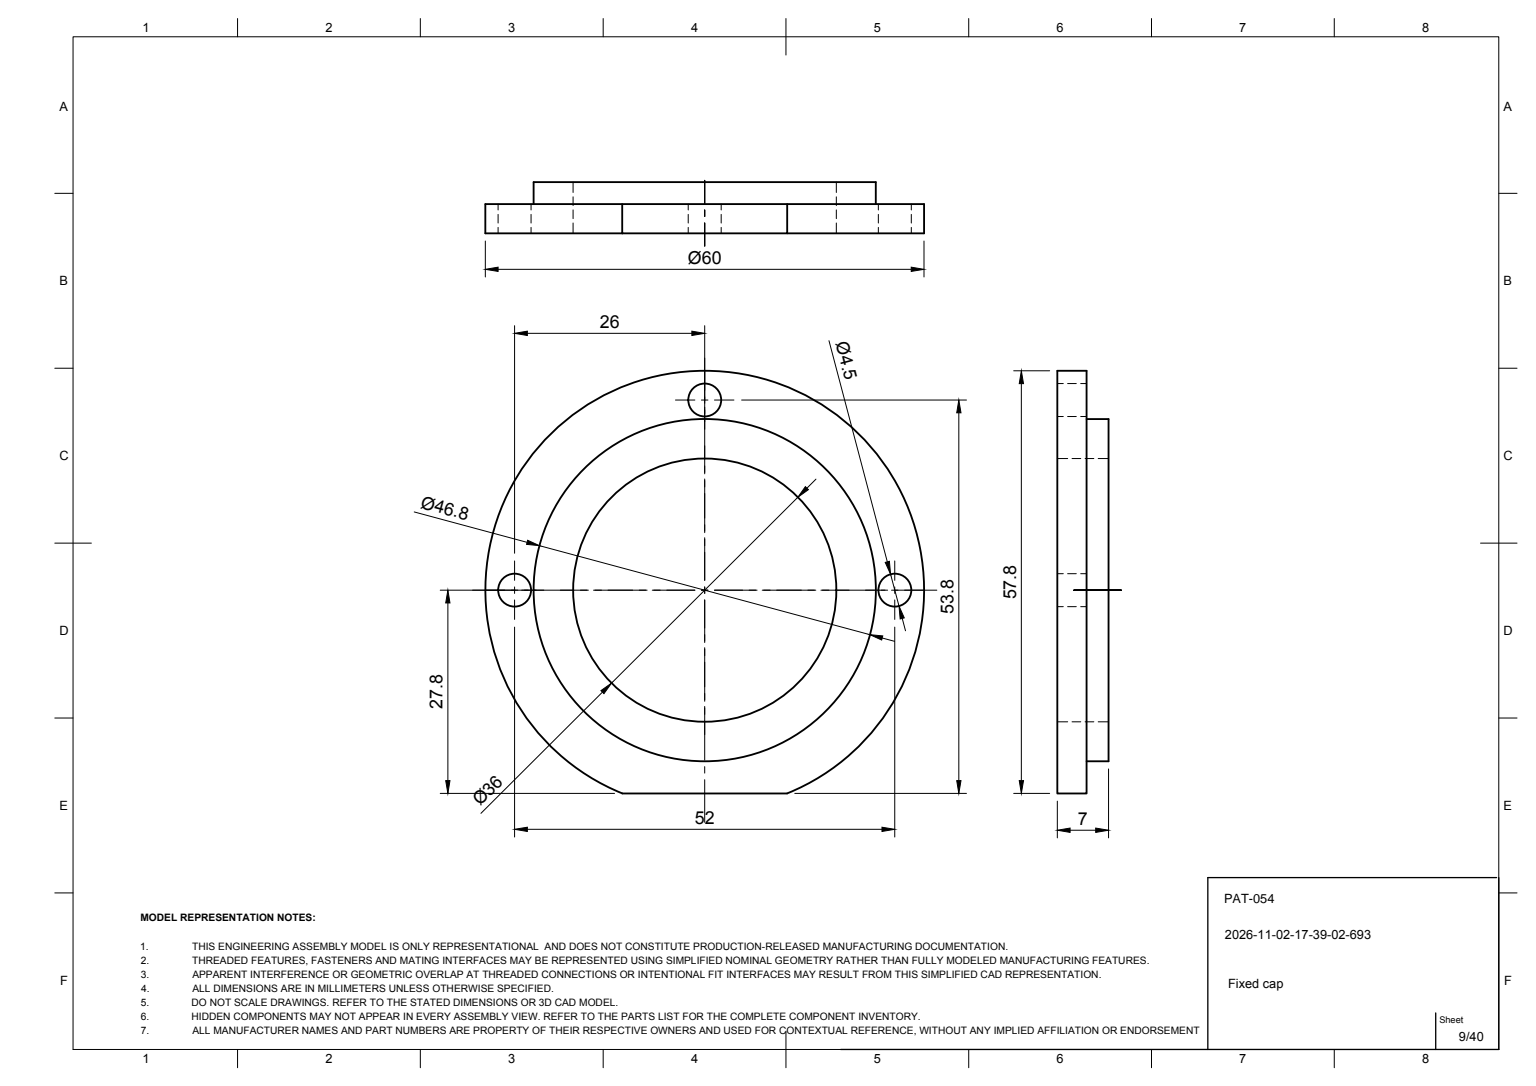
ISO-10303-21;
HEADER;
/* Generated by software containing ST-Developer
 * from STEP Tools, Inc. (www.steptools.com) 
 */

FILE_DESCRIPTION(
/* description */ ('PAT-054'),
/* implementation_level */ '2;1');

FILE_NAME(
/* name */ 'Fixed cap.step',
/* time_stamp */ '2026-10-29T16:38:13-07:00',
/* author */ (''),
/* organization */ (''),
/* preprocessor_version */ 'ST-DEVELOPER v20.2',
/* originating_system */ 'Autodesk Translation Framework v15.17.0.0',
/* authorisation */ '');

FILE_SCHEMA (('AUTOMOTIVE_DESIGN { 1 0 10303 214 3 1 1 }'));
ENDSEC;

DATA;
#10=MECHANICAL_DESIGN_GEOMETRIC_PRESENTATION_REPRESENTATION('',(#904),#33981);
#816=SHAPE_REPRESENTATION_RELATIONSHIP('SRR','None',#34189,#860);
#860=ADVANCED_BREP_SHAPE_REPRESENTATION('',(#963),#33937);
#904=STYLED_ITEM('',(#34531),#963);
#963=MANIFOLD_SOLID_BREP('Body1',#13015);
#1095=FACE_BOUND('',#2468,.T.);
#1096=FACE_BOUND('',#2469,.T.);
#1097=FACE_BOUND('',#2470,.T.);
#1098=FACE_BOUND('',#2471,.T.);
#1099=FACE_BOUND('',#2478,.T.);
#1100=FACE_BOUND('',#2481,.T.);
#1101=FACE_BOUND('',#2482,.T.);
#1102=FACE_BOUND('',#2483,.T.);
#1103=FACE_BOUND('',#2484,.T.);
#1265=PLANE('',#13748);
#1266=PLANE('',#13749);
#1267=PLANE('',#13765);
#1268=PLANE('',#13769);
#1660=FACE_OUTER_BOUND('',#2466,.T.);
#1661=FACE_OUTER_BOUND('',#2467,.T.);
#1662=FACE_OUTER_BOUND('',#2472,.T.);
#1663=FACE_OUTER_BOUND('',#2473,.T.);
#1664=FACE_OUTER_BOUND('',#2474,.T.);
#1665=FACE_OUTER_BOUND('',#2475,.T.);
#1666=FACE_OUTER_BOUND('',#2476,.T.);
#1667=FACE_OUTER_BOUND('',#2477,.T.);
#1668=FACE_OUTER_BOUND('',#2479,.T.);
#1669=FACE_OUTER_BOUND('',#2480,.T.);
#2466=EDGE_LOOP('',(#8873,#8874,#8875,#8876));
#2467=EDGE_LOOP('',(#8877,#8878));
#2468=EDGE_LOOP('',(#8879));
#2469=EDGE_LOOP('',(#8880));
#2470=EDGE_LOOP('',(#8881));
#2471=EDGE_LOOP('',(#8882));
#2472=EDGE_LOOP('',(#8883,#8884,#8885,#8886));
#2473=EDGE_LOOP('',(#8887,#8888,#8889,#8890));
#2474=EDGE_LOOP('',(#8891,#8892,#8893,#8894));
#2475=EDGE_LOOP('',(#8895,#8896,#8897,#8898));
#2476=EDGE_LOOP('',(#8899,#8900,#8901,#8902));
#2477=EDGE_LOOP('',(#8903));
#2478=EDGE_LOOP('',(#8904));
#2479=EDGE_LOOP('',(#8905,#8906,#8907,#8908));
#2480=EDGE_LOOP('',(#8909,#8910));
#2481=EDGE_LOOP('',(#8911));
#2482=EDGE_LOOP('',(#8912));
#2483=EDGE_LOOP('',(#8913));
#2484=EDGE_LOOP('',(#8914));
#3333=LINE('',#18902,#4267);
#3334=LINE('',#18904,#4268);
#3335=LINE('',#18906,#4269);
#3336=LINE('',#18907,#4270);
#3337=LINE('',#18922,#4271);
#3338=LINE('',#18926,#4272);
#3339=LINE('',#18930,#4273);
#3340=LINE('',#18934,#4274);
#3341=LINE('',#18942,#4275);
#4267=VECTOR('',#15366,1.);
#4268=VECTOR('',#15367,1.);
#4269=VECTOR('',#15368,1.);
#4270=VECTOR('',#15369,1.);
#4271=VECTOR('',#15388,0.225);
#4272=VECTOR('',#15393,0.225);
#4273=VECTOR('',#15398,0.225);
#4274=VECTOR('',#15403,2.34);
#4275=VECTOR('',#15414,1.8);
#5201=CIRCLE('',#13750,3.);
#5202=CIRCLE('',#13751,2.34);
#5203=CIRCLE('',#13752,0.225);
#5204=CIRCLE('',#13753,0.225);
#5205=CIRCLE('',#13754,0.225);
#5206=CIRCLE('',#13756,3.);
#5207=CIRCLE('',#13758,0.225);
#5208=CIRCLE('',#13760,0.225);
#5209=CIRCLE('',#13762,0.225);
#5210=CIRCLE('',#13764,2.34);
#5211=CIRCLE('',#13766,1.8);
#5212=CIRCLE('',#13768,1.8);
#5698=VERTEX_POINT('',#18900);
#5699=VERTEX_POINT('',#18901);
#5700=VERTEX_POINT('',#18903);
#5701=VERTEX_POINT('',#18905);
#5702=VERTEX_POINT('',#18910);
#5703=VERTEX_POINT('',#18912);
#5704=VERTEX_POINT('',#18914);
#5705=VERTEX_POINT('',#18916);
#5706=VERTEX_POINT('',#18921);
#5707=VERTEX_POINT('',#18925);
#5708=VERTEX_POINT('',#18929);
#5709=VERTEX_POINT('',#18933);
#5710=VERTEX_POINT('',#18937);
#5711=VERTEX_POINT('',#18940);
#6936=EDGE_CURVE('',#5698,#5699,#3333,.T.);
#6937=EDGE_CURVE('',#5700,#5698,#3334,.T.);
#6938=EDGE_CURVE('',#5701,#5700,#3335,.T.);
#6939=EDGE_CURVE('',#5699,#5701,#3336,.T.);
#6940=EDGE_CURVE('',#5700,#5698,#5201,.T.);
#6941=EDGE_CURVE('',#5702,#5702,#5202,.T.);
#6942=EDGE_CURVE('',#5703,#5703,#5203,.T.);
#6943=EDGE_CURVE('',#5704,#5704,#5204,.T.);
#6944=EDGE_CURVE('',#5705,#5705,#5205,.T.);
#6945=EDGE_CURVE('',#5701,#5699,#5206,.T.);
#6946=EDGE_CURVE('',#5705,#5706,#3337,.T.);
#6947=EDGE_CURVE('',#5706,#5706,#5207,.T.);
#6948=EDGE_CURVE('',#5704,#5707,#3338,.T.);
#6949=EDGE_CURVE('',#5707,#5707,#5208,.T.);
#6950=EDGE_CURVE('',#5703,#5708,#3339,.T.);
#6951=EDGE_CURVE('',#5708,#5708,#5209,.T.);
#6952=EDGE_CURVE('',#5702,#5709,#3340,.T.);
#6953=EDGE_CURVE('',#5709,#5709,#5210,.T.);
#6954=EDGE_CURVE('',#5710,#5710,#5211,.T.);
#6955=EDGE_CURVE('',#5711,#5711,#5212,.T.);
#6956=EDGE_CURVE('',#5711,#5710,#3341,.T.);
#8873=ORIENTED_EDGE('',*,*,#6936,.F.);
#8874=ORIENTED_EDGE('',*,*,#6937,.F.);
#8875=ORIENTED_EDGE('',*,*,#6938,.F.);
#8876=ORIENTED_EDGE('',*,*,#6939,.F.);
#8877=ORIENTED_EDGE('',*,*,#6937,.T.);
#8878=ORIENTED_EDGE('',*,*,#6940,.F.);
#8879=ORIENTED_EDGE('',*,*,#6941,.T.);
#8880=ORIENTED_EDGE('',*,*,#6942,.T.);
#8881=ORIENTED_EDGE('',*,*,#6943,.T.);
#8882=ORIENTED_EDGE('',*,*,#6944,.T.);
#8883=ORIENTED_EDGE('',*,*,#6938,.T.);
#8884=ORIENTED_EDGE('',*,*,#6940,.T.);
#8885=ORIENTED_EDGE('',*,*,#6936,.T.);
#8886=ORIENTED_EDGE('',*,*,#6945,.F.);
#8887=ORIENTED_EDGE('',*,*,#6944,.F.);
#8888=ORIENTED_EDGE('',*,*,#6946,.T.);
#8889=ORIENTED_EDGE('',*,*,#6947,.F.);
#8890=ORIENTED_EDGE('',*,*,#6946,.F.);
#8891=ORIENTED_EDGE('',*,*,#6943,.F.);
#8892=ORIENTED_EDGE('',*,*,#6948,.T.);
#8893=ORIENTED_EDGE('',*,*,#6949,.F.);
#8894=ORIENTED_EDGE('',*,*,#6948,.F.);
#8895=ORIENTED_EDGE('',*,*,#6942,.F.);
#8896=ORIENTED_EDGE('',*,*,#6950,.T.);
#8897=ORIENTED_EDGE('',*,*,#6951,.F.);
#8898=ORIENTED_EDGE('',*,*,#6950,.F.);
#8899=ORIENTED_EDGE('',*,*,#6941,.F.);
#8900=ORIENTED_EDGE('',*,*,#6952,.T.);
#8901=ORIENTED_EDGE('',*,*,#6953,.T.);
#8902=ORIENTED_EDGE('',*,*,#6952,.F.);
#8903=ORIENTED_EDGE('',*,*,#6953,.F.);
#8904=ORIENTED_EDGE('',*,*,#6954,.F.);
#8905=ORIENTED_EDGE('',*,*,#6955,.F.);
#8906=ORIENTED_EDGE('',*,*,#6956,.T.);
#8907=ORIENTED_EDGE('',*,*,#6954,.T.);
#8908=ORIENTED_EDGE('',*,*,#6956,.F.);
#8909=ORIENTED_EDGE('',*,*,#6939,.T.);
#8910=ORIENTED_EDGE('',*,*,#6945,.T.);
#8911=ORIENTED_EDGE('',*,*,#6947,.T.);
#8912=ORIENTED_EDGE('',*,*,#6949,.T.);
#8913=ORIENTED_EDGE('',*,*,#6951,.T.);
#8914=ORIENTED_EDGE('',*,*,#6955,.T.);
#12027=CYLINDRICAL_SURFACE('',#13755,3.);
#12028=CYLINDRICAL_SURFACE('',#13757,0.225);
#12029=CYLINDRICAL_SURFACE('',#13759,0.225);
#12030=CYLINDRICAL_SURFACE('',#13761,0.225);
#12031=CYLINDRICAL_SURFACE('',#13763,2.34);
#12032=CYLINDRICAL_SURFACE('',#13767,1.8);
#12372=ADVANCED_FACE('',(#1660),#1265,.F.);
#12373=ADVANCED_FACE('',(#1661,#1095,#1096,#1097,#1098),#1266,.F.);
#12374=ADVANCED_FACE('',(#1662),#12027,.T.);
#12375=ADVANCED_FACE('',(#1663),#12028,.F.);
#12376=ADVANCED_FACE('',(#1664),#12029,.F.);
#12377=ADVANCED_FACE('',(#1665),#12030,.F.);
#12378=ADVANCED_FACE('',(#1666),#12031,.T.);
#12379=ADVANCED_FACE('',(#1667,#1099),#1267,.F.);
#12380=ADVANCED_FACE('',(#1668),#12032,.F.);
#12381=ADVANCED_FACE('',(#1669,#1100,#1101,#1102,#1103),#1268,.T.);
#13015=CLOSED_SHELL('',(#12372,#12373,#12374,#12375,#12376,#12377,#12378,
#12379,#12380,#12381));
#13747=AXIS2_PLACEMENT_3D('',#18898,#15362,#15363);
#13748=AXIS2_PLACEMENT_3D('',#18899,#15364,#15365);
#13749=AXIS2_PLACEMENT_3D('',#18908,#15370,#15371);
#13750=AXIS2_PLACEMENT_3D('',#18909,#15372,#15373);
#13751=AXIS2_PLACEMENT_3D('',#18911,#15374,#15375);
#13752=AXIS2_PLACEMENT_3D('',#18913,#15376,#15377);
#13753=AXIS2_PLACEMENT_3D('',#18915,#15378,#15379);
#13754=AXIS2_PLACEMENT_3D('',#18917,#15380,#15381);
#13755=AXIS2_PLACEMENT_3D('',#18918,#15382,#15383);
#13756=AXIS2_PLACEMENT_3D('',#18919,#15384,#15385);
#13757=AXIS2_PLACEMENT_3D('',#18920,#15386,#15387);
#13758=AXIS2_PLACEMENT_3D('',#18923,#15389,#15390);
#13759=AXIS2_PLACEMENT_3D('',#18924,#15391,#15392);
#13760=AXIS2_PLACEMENT_3D('',#18927,#15394,#15395);
#13761=AXIS2_PLACEMENT_3D('',#18928,#15396,#15397);
#13762=AXIS2_PLACEMENT_3D('',#18931,#15399,#15400);
#13763=AXIS2_PLACEMENT_3D('',#18932,#15401,#15402);
#13764=AXIS2_PLACEMENT_3D('',#18935,#15404,#15405);
#13765=AXIS2_PLACEMENT_3D('',#18936,#15406,#15407);
#13766=AXIS2_PLACEMENT_3D('',#18938,#15408,#15409);
#13767=AXIS2_PLACEMENT_3D('',#18939,#15410,#15411);
#13768=AXIS2_PLACEMENT_3D('',#18941,#15412,#15413);
#13769=AXIS2_PLACEMENT_3D('',#18943,#15415,#15416);
#15362=DIRECTION('axis',(0.,0.,1.));
#15363=DIRECTION('refdir',(1.,0.,0.));
#15364=DIRECTION('center_axis',(0.,0.,1.));
#15365=DIRECTION('ref_axis',(0.,-1.,0.));
#15366=DIRECTION('',(1.,0.,0.));
#15367=DIRECTION('',(0.,-1.,0.));
#15368=DIRECTION('',(-1.,0.,0.));
#15369=DIRECTION('',(0.,1.,0.));
#15370=DIRECTION('center_axis',(1.,0.,0.));
#15371=DIRECTION('ref_axis',(0.,0.,-1.));
#15372=DIRECTION('center_axis',(1.,0.,0.));
#15373=DIRECTION('ref_axis',(0.,0.,-1.));
#15374=DIRECTION('center_axis',(1.,0.,0.));
#15375=DIRECTION('ref_axis',(0.,0.,-1.));
#15376=DIRECTION('center_axis',(1.,0.,0.));
#15377=DIRECTION('ref_axis',(0.,0.,-1.));
#15378=DIRECTION('center_axis',(1.,0.,0.));
#15379=DIRECTION('ref_axis',(0.,0.,-1.));
#15380=DIRECTION('center_axis',(1.,0.,0.));
#15381=DIRECTION('ref_axis',(0.,0.,-1.));
#15382=DIRECTION('center_axis',(1.,0.,0.));
#15383=DIRECTION('ref_axis',(0.,1.22464679914735E-16,1.));
#15384=DIRECTION('center_axis',(1.,0.,0.));
#15385=DIRECTION('ref_axis',(0.,0.,-1.));
#15386=DIRECTION('center_axis',(1.,0.,0.));
#15387=DIRECTION('ref_axis',(0.,0.,-1.));
#15388=DIRECTION('',(1.,0.,0.));
#15389=DIRECTION('center_axis',(-1.,0.,0.));
#15390=DIRECTION('ref_axis',(0.,0.,-1.));
#15391=DIRECTION('center_axis',(1.,0.,0.));
#15392=DIRECTION('ref_axis',(0.,0.,-1.));
#15393=DIRECTION('',(1.,0.,0.));
#15394=DIRECTION('center_axis',(-1.,0.,0.));
#15395=DIRECTION('ref_axis',(0.,0.,-1.));
#15396=DIRECTION('center_axis',(1.,0.,0.));
#15397=DIRECTION('ref_axis',(0.,0.,-1.));
#15398=DIRECTION('',(1.,0.,0.));
#15399=DIRECTION('center_axis',(-1.,0.,0.));
#15400=DIRECTION('ref_axis',(0.,0.,-1.));
#15401=DIRECTION('center_axis',(1.,0.,0.));
#15402=DIRECTION('ref_axis',(0.,0.,-1.));
#15403=DIRECTION('',(-1.,0.,0.));
#15404=DIRECTION('center_axis',(1.,0.,0.));
#15405=DIRECTION('ref_axis',(0.,0.,-1.));
#15406=DIRECTION('center_axis',(1.,0.,0.));
#15407=DIRECTION('ref_axis',(0.,0.,-1.));
#15408=DIRECTION('center_axis',(-1.,0.,0.));
#15409=DIRECTION('ref_axis',(0.,0.,-1.));
#15410=DIRECTION('center_axis',(1.,0.,0.));
#15411=DIRECTION('ref_axis',(0.,0.,-1.));
#15412=DIRECTION('center_axis',(-1.,0.,0.));
#15413=DIRECTION('ref_axis',(0.,0.,-1.));
#15414=DIRECTION('',(-1.,0.,0.));
#15415=DIRECTION('center_axis',(1.,0.,0.));
#15416=DIRECTION('ref_axis',(0.,0.,-1.));
#18898=CARTESIAN_POINT('',(0.,0.,0.));
#18899=CARTESIAN_POINT('Origin',(24.9,3.5,1.22));
#18900=CARTESIAN_POINT('',(25.,-1.12765242872084,1.22));
#18901=CARTESIAN_POINT('',(25.4,-1.12765242872084,1.22));
#18902=CARTESIAN_POINT('',(25.,-1.12765242872084,1.22));
#18903=CARTESIAN_POINT('',(25.,1.12765242872084,1.22));
#18904=CARTESIAN_POINT('',(25.,1.75,1.22));
#18905=CARTESIAN_POINT('',(25.4,1.12765242872084,1.22));
#18906=CARTESIAN_POINT('',(25.,1.12765242872084,1.22));
#18907=CARTESIAN_POINT('',(25.4,1.75,1.22));
#18908=CARTESIAN_POINT('Origin',(25.,0.,4.));
#18909=CARTESIAN_POINT('Origin',(25.,0.,4.));
#18910=CARTESIAN_POINT('',(25.,-2.86567351000481E-16,6.34));
#18911=CARTESIAN_POINT('Origin',(25.,0.,4.));
#18912=CARTESIAN_POINT('',(25.,-2.75545529808154E-17,6.825));
#18913=CARTESIAN_POINT('Origin',(25.,0.,6.6));
#18914=CARTESIAN_POINT('',(25.,2.6,4.225));
#18915=CARTESIAN_POINT('Origin',(25.,2.6,4.));
#18916=CARTESIAN_POINT('',(25.,-2.6,4.225));
#18917=CARTESIAN_POINT('Origin',(25.,-2.6,4.));
#18918=CARTESIAN_POINT('Origin',(25.,0.,4.));
#18919=CARTESIAN_POINT('Origin',(25.4,0.,4.));
#18920=CARTESIAN_POINT('Origin',(24.9,-2.6,4.));
#18921=CARTESIAN_POINT('',(25.4,-2.6,4.225));
#18922=CARTESIAN_POINT('',(24.9,-2.6,4.225));
#18923=CARTESIAN_POINT('Origin',(25.4,-2.6,4.));
#18924=CARTESIAN_POINT('Origin',(24.9,2.6,4.));
#18925=CARTESIAN_POINT('',(25.4,2.6,4.225));
#18926=CARTESIAN_POINT('',(24.9,2.6,4.225));
#18927=CARTESIAN_POINT('Origin',(25.4,2.6,4.));
#18928=CARTESIAN_POINT('Origin',(24.9,0.,6.6));
#18929=CARTESIAN_POINT('',(25.4,2.75545529808154E-17,6.825));
#18930=CARTESIAN_POINT('',(24.9,-2.75545529808154E-17,6.825));
#18931=CARTESIAN_POINT('Origin',(25.4,0.,6.6));
#18932=CARTESIAN_POINT('Origin',(24.7,0.,4.));
#18933=CARTESIAN_POINT('',(24.7,-2.86567351000481E-16,6.34));
#18934=CARTESIAN_POINT('',(24.7,-2.86567351000481E-16,6.34));
#18935=CARTESIAN_POINT('Origin',(24.7,0.,4.));
#18936=CARTESIAN_POINT('Origin',(24.7,0.,4.));
#18937=CARTESIAN_POINT('',(24.7,-2.20436423846524E-16,5.8));
#18938=CARTESIAN_POINT('Origin',(24.7,0.,4.));
#18939=CARTESIAN_POINT('Origin',(25.,0.,4.));
#18940=CARTESIAN_POINT('',(25.4,-2.20436423846524E-16,5.8));
#18941=CARTESIAN_POINT('Origin',(25.4,0.,4.));
#18942=CARTESIAN_POINT('',(25.,-2.20436423846524E-16,5.8));
#18943=CARTESIAN_POINT('Origin',(25.4,0.,4.));
#33885=UNCERTAINTY_MEASURE_WITH_UNIT(LENGTH_MEASURE(0.001),#33982,
'DISTANCE_ACCURACY_VALUE',
'Maximum model space distance between geometric entities at asserted c
onnectivities');
#33929=UNCERTAINTY_MEASURE_WITH_UNIT(LENGTH_MEASURE(0.001),#33982,
'DISTANCE_ACCURACY_VALUE',
'Maximum model space distance between geometric entities at asserted c
onnectivities');
#33937=(
GEOMETRIC_REPRESENTATION_CONTEXT(3)
GLOBAL_UNCERTAINTY_ASSIGNED_CONTEXT((#33885))
GLOBAL_UNIT_ASSIGNED_CONTEXT((#33982,#33984,#33985))
REPRESENTATION_CONTEXT('','3D')
);
#33981=(
GEOMETRIC_REPRESENTATION_CONTEXT(3)
GLOBAL_UNCERTAINTY_ASSIGNED_CONTEXT((#33929))
GLOBAL_UNIT_ASSIGNED_CONTEXT((#33982,#33984,#33985))
REPRESENTATION_CONTEXT('','3D')
);
#33982=(
LENGTH_UNIT()
NAMED_UNIT(*)
SI_UNIT(.CENTI.,.METRE.)
);
#33984=(
NAMED_UNIT(*)
PLANE_ANGLE_UNIT()
SI_UNIT($,.RADIAN.)
);
#33985=(
NAMED_UNIT(*)
SI_UNIT($,.STERADIAN.)
SOLID_ANGLE_UNIT()
);
#33993=SHAPE_DEFINITION_REPRESENTATION(#34044,#34189);
#34044=PRODUCT_DEFINITION_SHAPE('',$,#34241);
#34189=SHAPE_REPRESENTATION('',(#13747),#33937);
#34233=PRODUCT_DEFINITION_CONTEXT('part definition',#34388,'design');
#34241=PRODUCT_DEFINITION('Fixed cap','Fixed cap',#34292,#34233);
#34292=PRODUCT_DEFINITION_FORMATION('',$,#34397);
#34388=APPLICATION_CONTEXT(
'Core Data for Automotive Mechanical Design Process');
#34389=PRODUCT_CONTEXT('part definition',#34388,'mechanical');
#34397=PRODUCT('Fixed cap','Fixed cap','Fixed cap',(#34389));
#34525=COLOUR_RGB('Off White',0.89,0.88,0.83);
#34526=FILL_AREA_STYLE_COLOUR('',#34525);
#34527=FILL_AREA_STYLE('',(#34526));
#34528=SURFACE_STYLE_FILL_AREA(#34527);
#34529=SURFACE_SIDE_STYLE('',(#34528));
#34530=SURFACE_STYLE_USAGE(.BOTH.,#34529);
#34531=PRESENTATION_STYLE_ASSIGNMENT((#34530));
ENDSEC;
END-ISO-10303-21;
